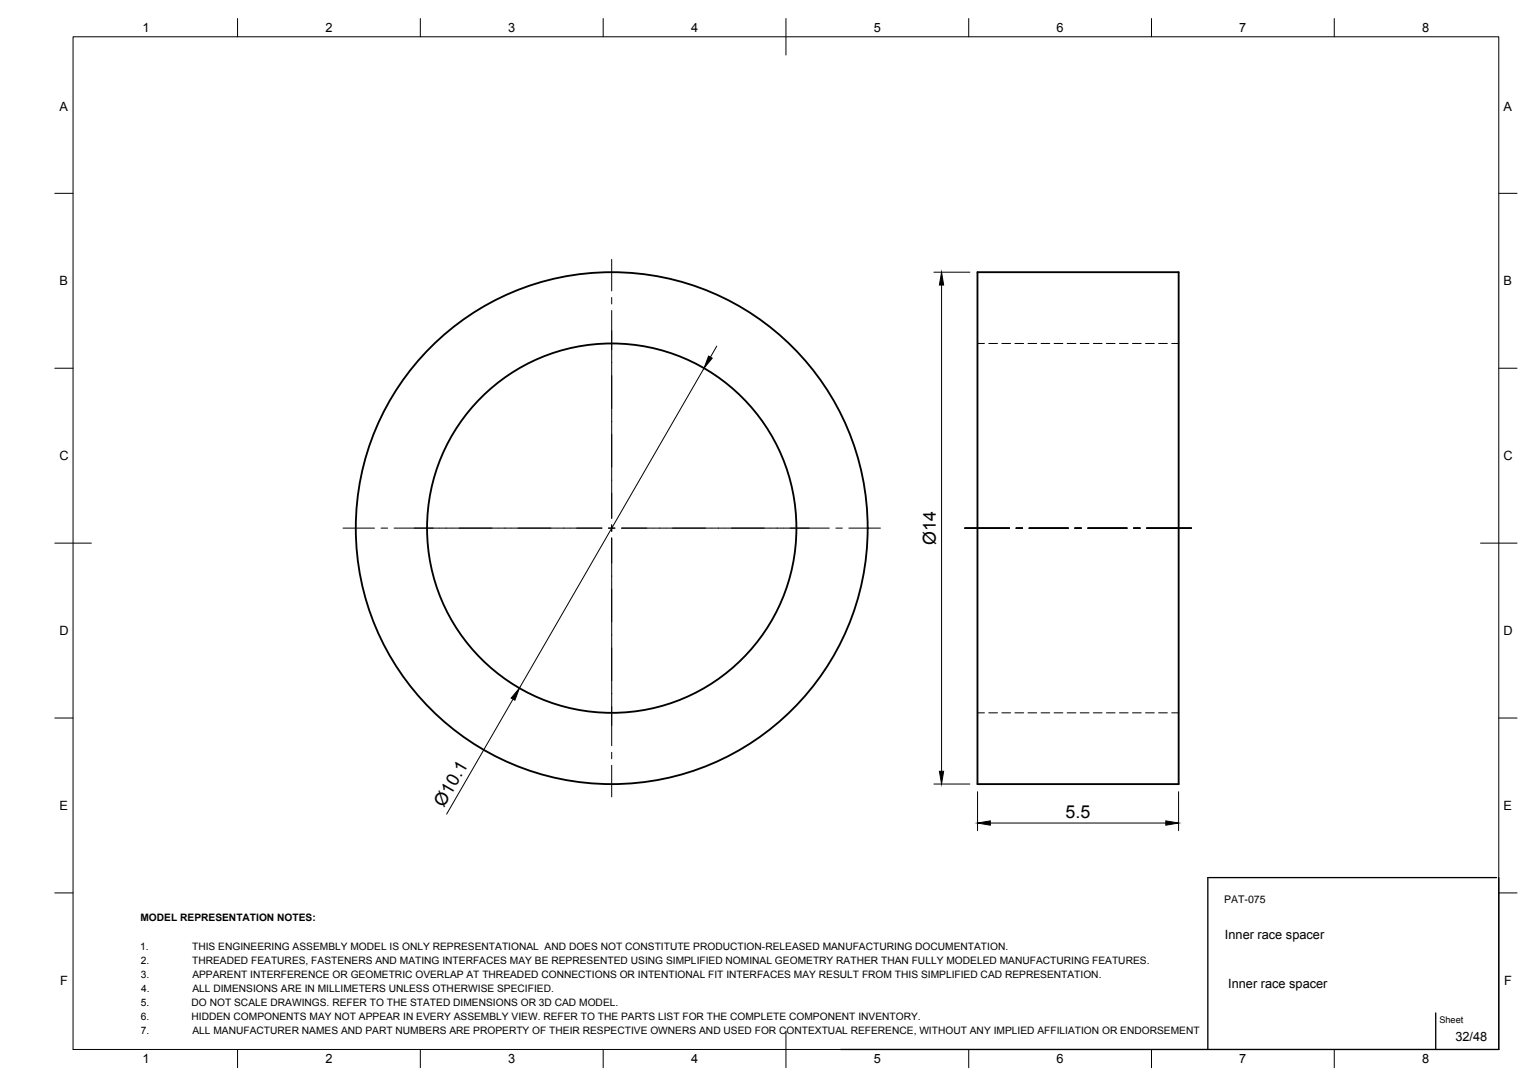
ISO-10303-21;
HEADER;
/* Generated by software containing ST-Developer
 * from STEP Tools, Inc. (www.steptools.com) 
 */

FILE_DESCRIPTION(
/* description */ ('Over-Centre Plunger Toggle Clamp on Slotted Fixture Frame'),
/* implementation_level */ '2;1');

FILE_NAME(
/* name */ 
'Inner race spacer.step',
/* time_stamp */ '2026-10-28T03:23:24-07:00',
/* author */ (''),
/* organization */ (''),
/* preprocessor_version */ 'ST-DEVELOPER v20.2',
/* originating_system */ 'Autodesk Translation Framework v15.17.0.0',
/* authorisation */ '');

FILE_SCHEMA (('AUTOMOTIVE_DESIGN { 1 0 10303 214 3 1 1 }'));
ENDSEC;

DATA;
#10=MECHANICAL_DESIGN_GEOMETRIC_PRESENTATION_REPRESENTATION('',(#546),#15212);
#454=SHAPE_REPRESENTATION_RELATIONSHIP('SRR','None',#15431,#496);
#496=ADVANCED_BREP_SHAPE_REPRESENTATION('',(#595),#15193);
#546=STYLED_ITEM('',(#15719),#595);
#595=MANIFOLD_SOLID_BREP('Body1',#8280);
#747=FACE_BOUND('',#2056,.T.);
#748=FACE_BOUND('',#2058,.T.);
#995=PLANE('',#9425);
#996=PLANE('',#9426);
#1431=FACE_OUTER_BOUND('',#2053,.T.);
#1432=FACE_OUTER_BOUND('',#2054,.T.);
#1433=FACE_OUTER_BOUND('',#2055,.T.);
#1434=FACE_OUTER_BOUND('',#2057,.T.);
#2053=EDGE_LOOP('',(#7085,#7086,#7087,#7088));
#2054=EDGE_LOOP('',(#7089,#7090,#7091,#7092));
#2055=EDGE_LOOP('',(#7093));
#2056=EDGE_LOOP('',(#7094));
#2057=EDGE_LOOP('',(#7095));
#2058=EDGE_LOOP('',(#7096));
#2697=LINE('',#14360,#3327);
#2698=LINE('',#14366,#3328);
#3327=VECTOR('',#11536,0.505);
#3328=VECTOR('',#11543,0.7);
#3763=CIRCLE('',#9420,0.505);
#3764=CIRCLE('',#9421,0.505);
#3765=CIRCLE('',#9423,0.7);
#3766=CIRCLE('',#9424,0.7);
#4371=VERTEX_POINT('',#14357);
#4372=VERTEX_POINT('',#14359);
#4373=VERTEX_POINT('',#14363);
#4374=VERTEX_POINT('',#14365);
#5303=EDGE_CURVE('',#4371,#4371,#3763,.T.);
#5304=EDGE_CURVE('',#4371,#4372,#2697,.T.);
#5305=EDGE_CURVE('',#4372,#4372,#3764,.T.);
#5306=EDGE_CURVE('',#4373,#4373,#3765,.T.);
#5307=EDGE_CURVE('',#4373,#4374,#2698,.T.);
#5308=EDGE_CURVE('',#4374,#4374,#3766,.T.);
#7085=ORIENTED_EDGE('',*,*,#5303,.F.);
#7086=ORIENTED_EDGE('',*,*,#5304,.T.);
#7087=ORIENTED_EDGE('',*,*,#5305,.T.);
#7088=ORIENTED_EDGE('',*,*,#5304,.F.);
#7089=ORIENTED_EDGE('',*,*,#5306,.F.);
#7090=ORIENTED_EDGE('',*,*,#5307,.T.);
#7091=ORIENTED_EDGE('',*,*,#5308,.T.);
#7092=ORIENTED_EDGE('',*,*,#5307,.F.);
#7093=ORIENTED_EDGE('',*,*,#5306,.T.);
#7094=ORIENTED_EDGE('',*,*,#5303,.T.);
#7095=ORIENTED_EDGE('',*,*,#5308,.F.);
#7096=ORIENTED_EDGE('',*,*,#5305,.F.);
#7719=CYLINDRICAL_SURFACE('',#9419,0.505);
#7720=CYLINDRICAL_SURFACE('',#9422,0.7);
#8103=ADVANCED_FACE('',(#1431),#7719,.F.);
#8104=ADVANCED_FACE('',(#1432),#7720,.T.);
#8105=ADVANCED_FACE('',(#1433,#747),#995,.T.);
#8106=ADVANCED_FACE('',(#1434,#748),#996,.F.);
#8280=CLOSED_SHELL('',(#8103,#8104,#8105,#8106));
#9418=AXIS2_PLACEMENT_3D('',#14355,#11530,#11531);
#9419=AXIS2_PLACEMENT_3D('',#14356,#11532,#11533);
#9420=AXIS2_PLACEMENT_3D('',#14358,#11534,#11535);
#9421=AXIS2_PLACEMENT_3D('',#14361,#11537,#11538);
#9422=AXIS2_PLACEMENT_3D('',#14362,#11539,#11540);
#9423=AXIS2_PLACEMENT_3D('',#14364,#11541,#11542);
#9424=AXIS2_PLACEMENT_3D('',#14367,#11544,#11545);
#9425=AXIS2_PLACEMENT_3D('',#14368,#11546,#11547);
#9426=AXIS2_PLACEMENT_3D('',#14369,#11548,#11549);
#11530=DIRECTION('axis',(0.,0.,1.));
#11531=DIRECTION('refdir',(1.,0.,0.));
#11532=DIRECTION('center_axis',(0.,1.,0.));
#11533=DIRECTION('ref_axis',(1.,0.,0.));
#11534=DIRECTION('center_axis',(0.,-1.,0.));
#11535=DIRECTION('ref_axis',(1.,0.,0.));
#11536=DIRECTION('',(0.,-1.,0.));
#11537=DIRECTION('center_axis',(0.,-1.,0.));
#11538=DIRECTION('ref_axis',(1.,0.,0.));
#11539=DIRECTION('center_axis',(0.,1.,0.));
#11540=DIRECTION('ref_axis',(1.,0.,0.));
#11541=DIRECTION('center_axis',(0.,1.,0.));
#11542=DIRECTION('ref_axis',(1.,0.,0.));
#11543=DIRECTION('',(0.,-1.,0.));
#11544=DIRECTION('center_axis',(0.,1.,0.));
#11545=DIRECTION('ref_axis',(1.,0.,0.));
#11546=DIRECTION('center_axis',(0.,1.,0.));
#11547=DIRECTION('ref_axis',(1.,0.,0.));
#11548=DIRECTION('center_axis',(0.,1.,0.));
#11549=DIRECTION('ref_axis',(1.,0.,0.));
#14355=CARTESIAN_POINT('',(0.,0.,0.));
#14356=CARTESIAN_POINT('Origin',(-4.,0.45,11.));
#14357=CARTESIAN_POINT('',(-4.505,1.,11.));
#14358=CARTESIAN_POINT('Origin',(-4.,1.,11.));
#14359=CARTESIAN_POINT('',(-4.505,0.45,11.));
#14360=CARTESIAN_POINT('',(-4.505,0.45,11.));
#14361=CARTESIAN_POINT('Origin',(-4.,0.45,11.));
#14362=CARTESIAN_POINT('Origin',(-4.,0.45,11.));
#14363=CARTESIAN_POINT('',(-4.7,1.,11.));
#14364=CARTESIAN_POINT('Origin',(-4.,1.,11.));
#14365=CARTESIAN_POINT('',(-4.7,0.45,11.));
#14366=CARTESIAN_POINT('',(-4.7,0.45,11.));
#14367=CARTESIAN_POINT('Origin',(-4.,0.45,11.));
#14368=CARTESIAN_POINT('Origin',(-4.,1.,11.));
#14369=CARTESIAN_POINT('Origin',(-4.,0.45,11.));
#15143=UNCERTAINTY_MEASURE_WITH_UNIT(LENGTH_MEASURE(0.001),#15213,
'DISTANCE_ACCURACY_VALUE',
'Maximum model space distance between geometric entities at asserted c
onnectivities');
#15162=UNCERTAINTY_MEASURE_WITH_UNIT(LENGTH_MEASURE(0.001),#15213,
'DISTANCE_ACCURACY_VALUE',
'Maximum model space distance between geometric entities at asserted c
onnectivities');
#15193=(
GEOMETRIC_REPRESENTATION_CONTEXT(3)
GLOBAL_UNCERTAINTY_ASSIGNED_CONTEXT((#15143))
GLOBAL_UNIT_ASSIGNED_CONTEXT((#15213,#15215,#15216))
REPRESENTATION_CONTEXT('','3D')
);
#15212=(
GEOMETRIC_REPRESENTATION_CONTEXT(3)
GLOBAL_UNCERTAINTY_ASSIGNED_CONTEXT((#15162))
GLOBAL_UNIT_ASSIGNED_CONTEXT((#15213,#15215,#15216))
REPRESENTATION_CONTEXT('','3D')
);
#15213=(
LENGTH_UNIT()
NAMED_UNIT(*)
SI_UNIT(.CENTI.,.METRE.)
);
#15215=(
NAMED_UNIT(*)
PLANE_ANGLE_UNIT()
SI_UNIT($,.RADIAN.)
);
#15216=(
NAMED_UNIT(*)
SI_UNIT($,.STERADIAN.)
SOLID_ANGLE_UNIT()
);
#15247=SHAPE_DEFINITION_REPRESENTATION(#15303,#15431);
#15303=PRODUCT_DEFINITION_SHAPE('',$,#15481);
#15431=SHAPE_REPRESENTATION('',(#9418),#15193);
#15450=PRODUCT_DEFINITION_CONTEXT('part definition',#15599,'design');
#15481=PRODUCT_DEFINITION('Inner race spacer','Inner race spacer',#15530,
#15450);
#15530=PRODUCT_DEFINITION_FORMATION('',$,#15631);
#15599=APPLICATION_CONTEXT(
'Core Data for Automotive Mechanical Design Process');
#15600=PRODUCT_CONTEXT('part definition',#15599,'mechanical');
#15631=PRODUCT('Inner race spacer','Inner race spacer',
'Inner race spacer',(#15600));
#15713=COLOUR_RGB('Grey',0.48,0.52,0.57);
#15714=FILL_AREA_STYLE_COLOUR('',#15713);
#15715=FILL_AREA_STYLE('',(#15714));
#15716=SURFACE_STYLE_FILL_AREA(#15715);
#15717=SURFACE_SIDE_STYLE('',(#15716));
#15718=SURFACE_STYLE_USAGE(.BOTH.,#15717);
#15719=PRESENTATION_STYLE_ASSIGNMENT((#15718));
ENDSEC;
END-ISO-10303-21;
